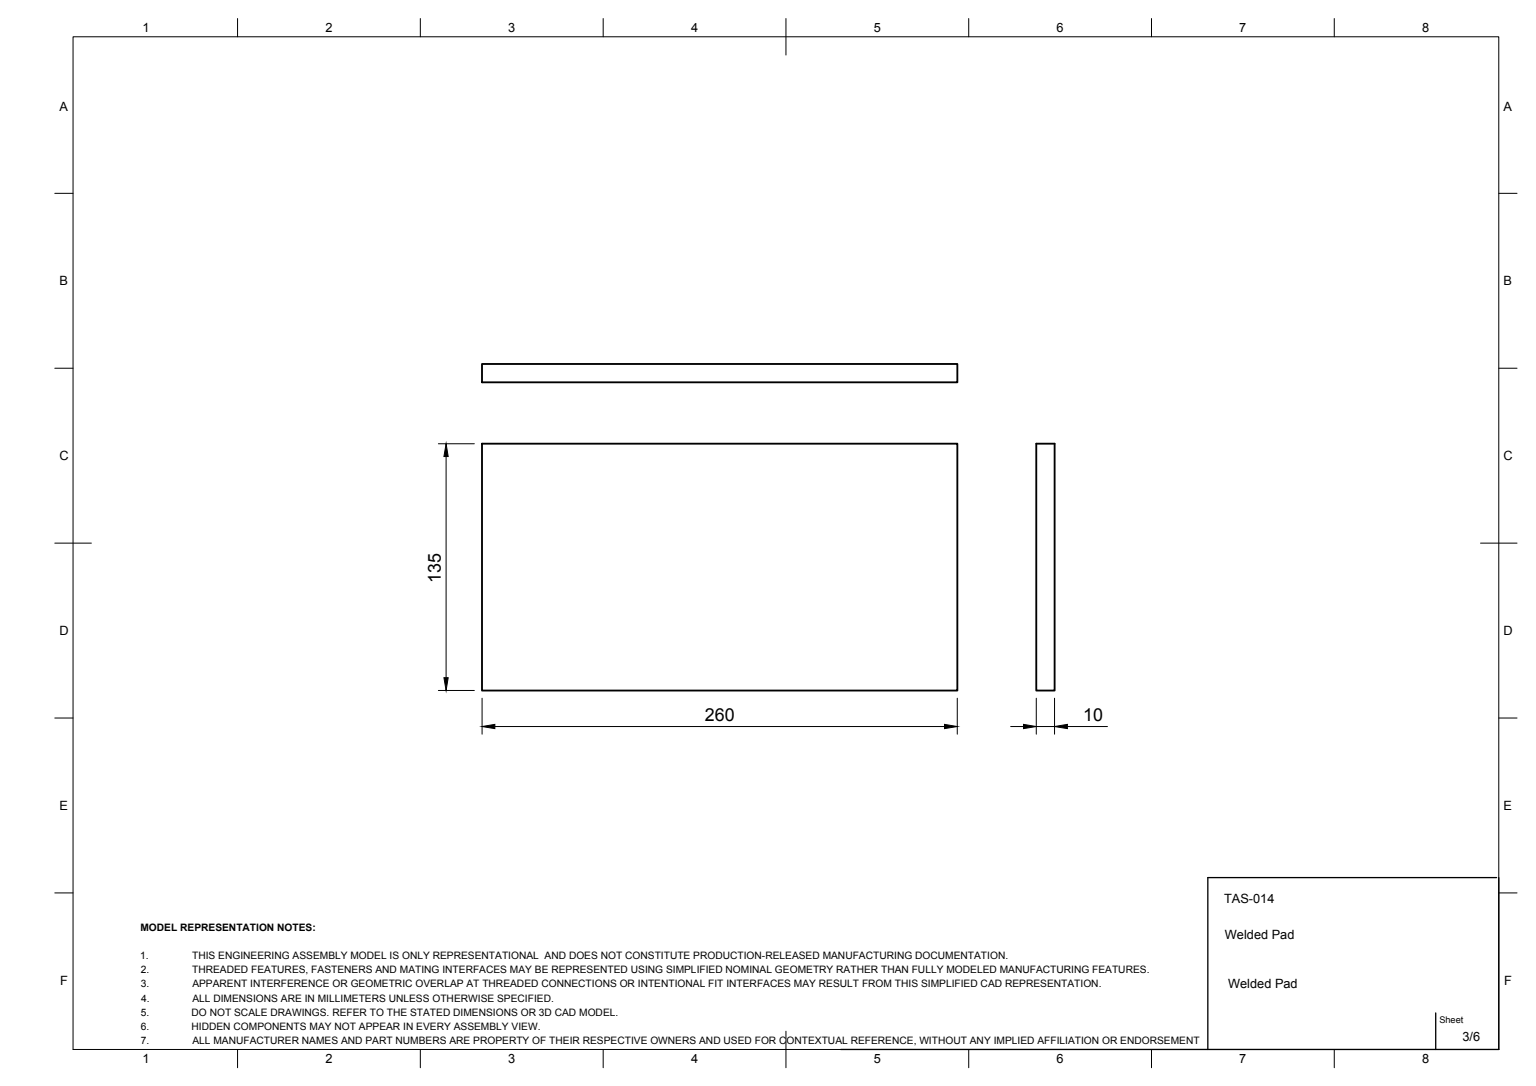
ISO-10303-21;
HEADER;
/* Generated by software containing ST-Developer
 * from STEP Tools, Inc. (www.steptools.com) 
 */

FILE_DESCRIPTION(
/* description */ ('STEP AP214'),
/* implementation_level */ '2;1');

FILE_NAME(
/* name */ 'Welded Pad.step',
/* time_stamp */ '2026-11-15T15:22:30-08:00',
/* author */ (''),
/* organization */ (''),
/* preprocessor_version */ 'ST-DEVELOPER v20.2',
/* originating_system */ 'Autodesk Translation Framework v15.17.0.0',
/* authorisation */ '');

FILE_SCHEMA (('AUTOMOTIVE_DESIGN { 1 0 10303 214 3 1 1 }'));
ENDSEC;

DATA;
#10=MECHANICAL_DESIGN_GEOMETRIC_PRESENTATION_REPRESENTATION('',(#85),#3119);
#68=SHAPE_REPRESENTATION_RELATIONSHIP('SRR','None',#3150,#72);
#72=ADVANCED_BREP_SHAPE_REPRESENTATION('',(#92),#3116);
#85=STYLED_ITEM('',(#3178),#92);
#92=MANIFOLD_SOLID_BREP('Body1',#1804);
#281=FACE_OUTER_BOUND('',#382,.T.);
#282=FACE_OUTER_BOUND('',#383,.T.);
#283=FACE_OUTER_BOUND('',#384,.T.);
#284=FACE_OUTER_BOUND('',#385,.T.);
#285=FACE_OUTER_BOUND('',#386,.T.);
#286=FACE_OUTER_BOUND('',#387,.T.);
#382=EDGE_LOOP('',(#1568,#1569,#1570,#1571));
#383=EDGE_LOOP('',(#1572,#1573,#1574,#1575));
#384=EDGE_LOOP('',(#1576,#1577,#1578,#1579));
#385=EDGE_LOOP('',(#1580,#1581,#1582,#1583));
#386=EDGE_LOOP('',(#1584,#1585,#1586,#1587));
#387=EDGE_LOOP('',(#1588,#1589,#1590,#1591));
#537=LINE('',#3011,#712);
#538=LINE('',#3013,#713);
#539=LINE('',#3015,#714);
#540=LINE('',#3016,#715);
#541=LINE('',#3019,#716);
#542=LINE('',#3021,#717);
#543=LINE('',#3022,#718);
#544=LINE('',#3025,#719);
#545=LINE('',#3027,#720);
#546=LINE('',#3028,#721);
#547=LINE('',#3030,#722);
#548=LINE('',#3031,#723);
#712=VECTOR('',#2472,1000.);
#713=VECTOR('',#2473,1000.);
#714=VECTOR('',#2474,1000.);
#715=VECTOR('',#2475,1000.);
#716=VECTOR('',#2478,1000.);
#717=VECTOR('',#2479,1000.);
#718=VECTOR('',#2480,1000.);
#719=VECTOR('',#2483,1000.);
#720=VECTOR('',#2484,1000.);
#721=VECTOR('',#2485,1000.);
#722=VECTOR('',#2488,1000.);
#723=VECTOR('',#2489,1000.);
#895=VERTEX_POINT('',#3009);
#896=VERTEX_POINT('',#3010);
#897=VERTEX_POINT('',#3012);
#898=VERTEX_POINT('',#3014);
#899=VERTEX_POINT('',#3018);
#900=VERTEX_POINT('',#3020);
#901=VERTEX_POINT('',#3024);
#902=VERTEX_POINT('',#3026);
#1129=EDGE_CURVE('',#895,#896,#537,.T.);
#1130=EDGE_CURVE('',#897,#896,#538,.T.);
#1131=EDGE_CURVE('',#898,#897,#539,.T.);
#1132=EDGE_CURVE('',#898,#895,#540,.T.);
#1133=EDGE_CURVE('',#896,#899,#541,.T.);
#1134=EDGE_CURVE('',#900,#899,#542,.T.);
#1135=EDGE_CURVE('',#897,#900,#543,.T.);
#1136=EDGE_CURVE('',#899,#901,#544,.T.);
#1137=EDGE_CURVE('',#902,#901,#545,.T.);
#1138=EDGE_CURVE('',#900,#902,#546,.T.);
#1139=EDGE_CURVE('',#901,#895,#547,.T.);
#1140=EDGE_CURVE('',#902,#898,#548,.T.);
#1568=ORIENTED_EDGE('',*,*,#1129,.T.);
#1569=ORIENTED_EDGE('',*,*,#1130,.F.);
#1570=ORIENTED_EDGE('',*,*,#1131,.F.);
#1571=ORIENTED_EDGE('',*,*,#1132,.T.);
#1572=ORIENTED_EDGE('',*,*,#1133,.T.);
#1573=ORIENTED_EDGE('',*,*,#1134,.F.);
#1574=ORIENTED_EDGE('',*,*,#1135,.F.);
#1575=ORIENTED_EDGE('',*,*,#1130,.T.);
#1576=ORIENTED_EDGE('',*,*,#1136,.T.);
#1577=ORIENTED_EDGE('',*,*,#1137,.F.);
#1578=ORIENTED_EDGE('',*,*,#1138,.F.);
#1579=ORIENTED_EDGE('',*,*,#1134,.T.);
#1580=ORIENTED_EDGE('',*,*,#1139,.T.);
#1581=ORIENTED_EDGE('',*,*,#1132,.F.);
#1582=ORIENTED_EDGE('',*,*,#1140,.F.);
#1583=ORIENTED_EDGE('',*,*,#1137,.T.);
#1584=ORIENTED_EDGE('',*,*,#1131,.T.);
#1585=ORIENTED_EDGE('',*,*,#1135,.T.);
#1586=ORIENTED_EDGE('',*,*,#1138,.T.);
#1587=ORIENTED_EDGE('',*,*,#1140,.T.);
#1588=ORIENTED_EDGE('',*,*,#1129,.F.);
#1589=ORIENTED_EDGE('',*,*,#1139,.F.);
#1590=ORIENTED_EDGE('',*,*,#1136,.F.);
#1591=ORIENTED_EDGE('',*,*,#1133,.F.);
#1688=PLANE('',#2001);
#1689=PLANE('',#2002);
#1690=PLANE('',#2003);
#1691=PLANE('',#2004);
#1692=PLANE('',#2005);
#1693=PLANE('',#2006);
#1781=ADVANCED_FACE('',(#281),#1688,.F.);
#1782=ADVANCED_FACE('',(#282),#1689,.F.);
#1783=ADVANCED_FACE('',(#283),#1690,.F.);
#1784=ADVANCED_FACE('',(#284),#1691,.F.);
#1785=ADVANCED_FACE('',(#285),#1692,.T.);
#1786=ADVANCED_FACE('',(#286),#1693,.F.);
#1804=CLOSED_SHELL('',(#1781,#1782,#1783,#1784,#1785,#1786));
#2000=AXIS2_PLACEMENT_3D('',#3007,#2468,#2469);
#2001=AXIS2_PLACEMENT_3D('',#3008,#2470,#2471);
#2002=AXIS2_PLACEMENT_3D('',#3017,#2476,#2477);
#2003=AXIS2_PLACEMENT_3D('',#3023,#2481,#2482);
#2004=AXIS2_PLACEMENT_3D('',#3029,#2486,#2487);
#2005=AXIS2_PLACEMENT_3D('',#3032,#2490,#2491);
#2006=AXIS2_PLACEMENT_3D('',#3033,#2492,#2493);
#2468=DIRECTION('axis',(0.,0.,1.));
#2469=DIRECTION('refdir',(1.,0.,0.));
#2470=DIRECTION('center_axis',(-1.,-1.06752213906265E-16,0.));
#2471=DIRECTION('ref_axis',(1.06752213906265E-16,-1.,0.));
#2472=DIRECTION('',(-1.06752213906265E-16,1.,0.));
#2473=DIRECTION('',(0.,0.,-1.));
#2474=DIRECTION('',(-1.06752213906265E-16,1.,0.));
#2475=DIRECTION('',(0.,0.,-1.));
#2476=DIRECTION('center_axis',(0.,-1.,0.));
#2477=DIRECTION('ref_axis',(0.,0.,-1.));
#2478=DIRECTION('',(-1.,0.,0.));
#2479=DIRECTION('',(0.,0.,-1.));
#2480=DIRECTION('',(-1.,0.,0.));
#2481=DIRECTION('center_axis',(1.,1.06752213906265E-16,0.));
#2482=DIRECTION('ref_axis',(-1.06752213906265E-16,1.,0.));
#2483=DIRECTION('',(1.06752213906265E-16,-1.,0.));
#2484=DIRECTION('',(0.,0.,-1.));
#2485=DIRECTION('',(1.06752213906265E-16,-1.,0.));
#2486=DIRECTION('center_axis',(0.,1.,0.));
#2487=DIRECTION('ref_axis',(0.,0.,1.));
#2488=DIRECTION('',(1.,0.,0.));
#2489=DIRECTION('',(1.,0.,0.));
#2490=DIRECTION('center_axis',(0.,0.,1.));
#2491=DIRECTION('ref_axis',(1.,0.,0.));
#2492=DIRECTION('center_axis',(0.,0.,1.));
#2493=DIRECTION('ref_axis',(1.,0.,0.));
#3007=CARTESIAN_POINT('',(0.,0.,0.));
#3008=CARTESIAN_POINT('Origin',(67.5,130.,5.));
#3009=CARTESIAN_POINT('',(67.5,-130.,-5.));
#3010=CARTESIAN_POINT('',(67.5,130.,-5.));
#3011=CARTESIAN_POINT('',(67.5,130.,-5.));
#3012=CARTESIAN_POINT('',(67.5,130.,5.));
#3013=CARTESIAN_POINT('',(67.5,130.,5.));
#3014=CARTESIAN_POINT('',(67.5,-130.,5.));
#3015=CARTESIAN_POINT('',(67.5,130.,5.));
#3016=CARTESIAN_POINT('',(67.5,-130.,5.));
#3017=CARTESIAN_POINT('Origin',(-67.5,130.,5.));
#3018=CARTESIAN_POINT('',(-67.5,130.,-5.));
#3019=CARTESIAN_POINT('',(-67.5,130.,-5.));
#3020=CARTESIAN_POINT('',(-67.5,130.,5.));
#3021=CARTESIAN_POINT('',(-67.5,130.,5.));
#3022=CARTESIAN_POINT('',(-67.5,130.,5.));
#3023=CARTESIAN_POINT('Origin',(-67.5,130.,5.));
#3024=CARTESIAN_POINT('',(-67.5,-130.,-5.));
#3025=CARTESIAN_POINT('',(-67.5,130.,-5.));
#3026=CARTESIAN_POINT('',(-67.5,-130.,5.));
#3027=CARTESIAN_POINT('',(-67.5,-130.,5.));
#3028=CARTESIAN_POINT('',(-67.5,130.,5.));
#3029=CARTESIAN_POINT('Origin',(-67.5,-130.,5.));
#3030=CARTESIAN_POINT('',(-67.5,-130.,-5.));
#3031=CARTESIAN_POINT('',(-67.5,-130.,5.));
#3032=CARTESIAN_POINT('Origin',(0.,0.,5.));
#3033=CARTESIAN_POINT('Origin',(0.,0.,-5.));
#3110=UNCERTAINTY_MEASURE_WITH_UNIT(LENGTH_MEASURE(0.01),#3120,
'DISTANCE_ACCURACY_VALUE',
'Maximum model space distance between geometric entities at asserted c
onnectivities');
#3113=UNCERTAINTY_MEASURE_WITH_UNIT(LENGTH_MEASURE(0.01),#3120,
'DISTANCE_ACCURACY_VALUE',
'Maximum model space distance between geometric entities at asserted c
onnectivities');
#3116=(
GEOMETRIC_REPRESENTATION_CONTEXT(3)
GLOBAL_UNCERTAINTY_ASSIGNED_CONTEXT((#3110))
GLOBAL_UNIT_ASSIGNED_CONTEXT((#3120,#3122,#3123))
REPRESENTATION_CONTEXT('','3D')
);
#3119=(
GEOMETRIC_REPRESENTATION_CONTEXT(3)
GLOBAL_UNCERTAINTY_ASSIGNED_CONTEXT((#3113))
GLOBAL_UNIT_ASSIGNED_CONTEXT((#3120,#3122,#3123))
REPRESENTATION_CONTEXT('','3D')
);
#3120=(
LENGTH_UNIT()
NAMED_UNIT(*)
SI_UNIT(.MILLI.,.METRE.)
);
#3122=(
NAMED_UNIT(*)
PLANE_ANGLE_UNIT()
SI_UNIT($,.RADIAN.)
);
#3123=(
NAMED_UNIT(*)
SI_UNIT($,.STERADIAN.)
SOLID_ANGLE_UNIT()
);
#3126=SHAPE_DEFINITION_REPRESENTATION(#3131,#3150);
#3131=PRODUCT_DEFINITION_SHAPE('',$,#3156);
#3150=SHAPE_REPRESENTATION('',(#2000),#3116);
#3153=PRODUCT_DEFINITION_CONTEXT('part definition',#3170,'design');
#3156=PRODUCT_DEFINITION('Welded Pad','Welded Pad',#3161,#3153);
#3161=PRODUCT_DEFINITION_FORMATION('',$,#3174);
#3170=APPLICATION_CONTEXT(
'Core Data for Automotive Mechanical Design Process');
#3171=PRODUCT_CONTEXT('part definition',#3170,'mechanical');
#3174=PRODUCT('Welded Pad','Welded Pad',$,(#3171));
#3178=PRESENTATION_STYLE_ASSIGNMENT((#3180));
#3180=SURFACE_STYLE_USAGE(.BOTH.,#3182);
#3182=SURFACE_SIDE_STYLE('',(#3184));
#3184=SURFACE_STYLE_FILL_AREA(#3186);
#3186=FILL_AREA_STYLE('Opaque(202,209,238)',(#3188));
#3188=FILL_AREA_STYLE_COLOUR('Opaque(202,209,238)',#3190);
#3190=COLOUR_RGB('Opaque(202,209,238)',0.792156862745098,0.819607843137255,
0.933333333333333);
ENDSEC;
END-ISO-10303-21;
